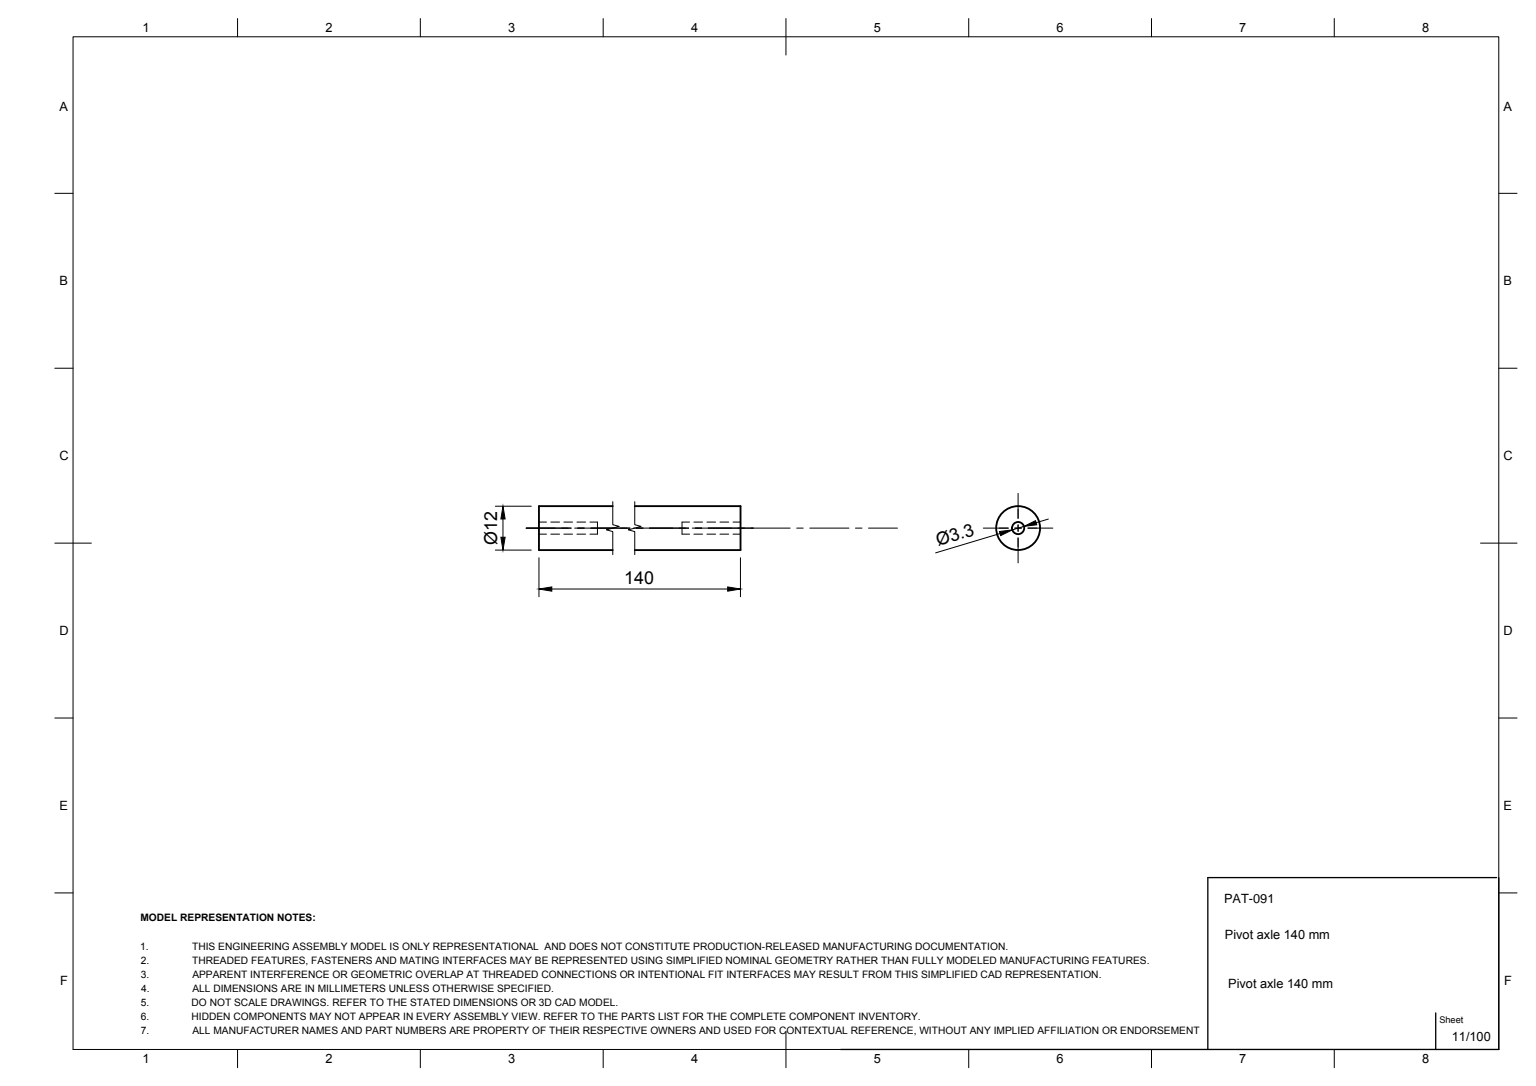
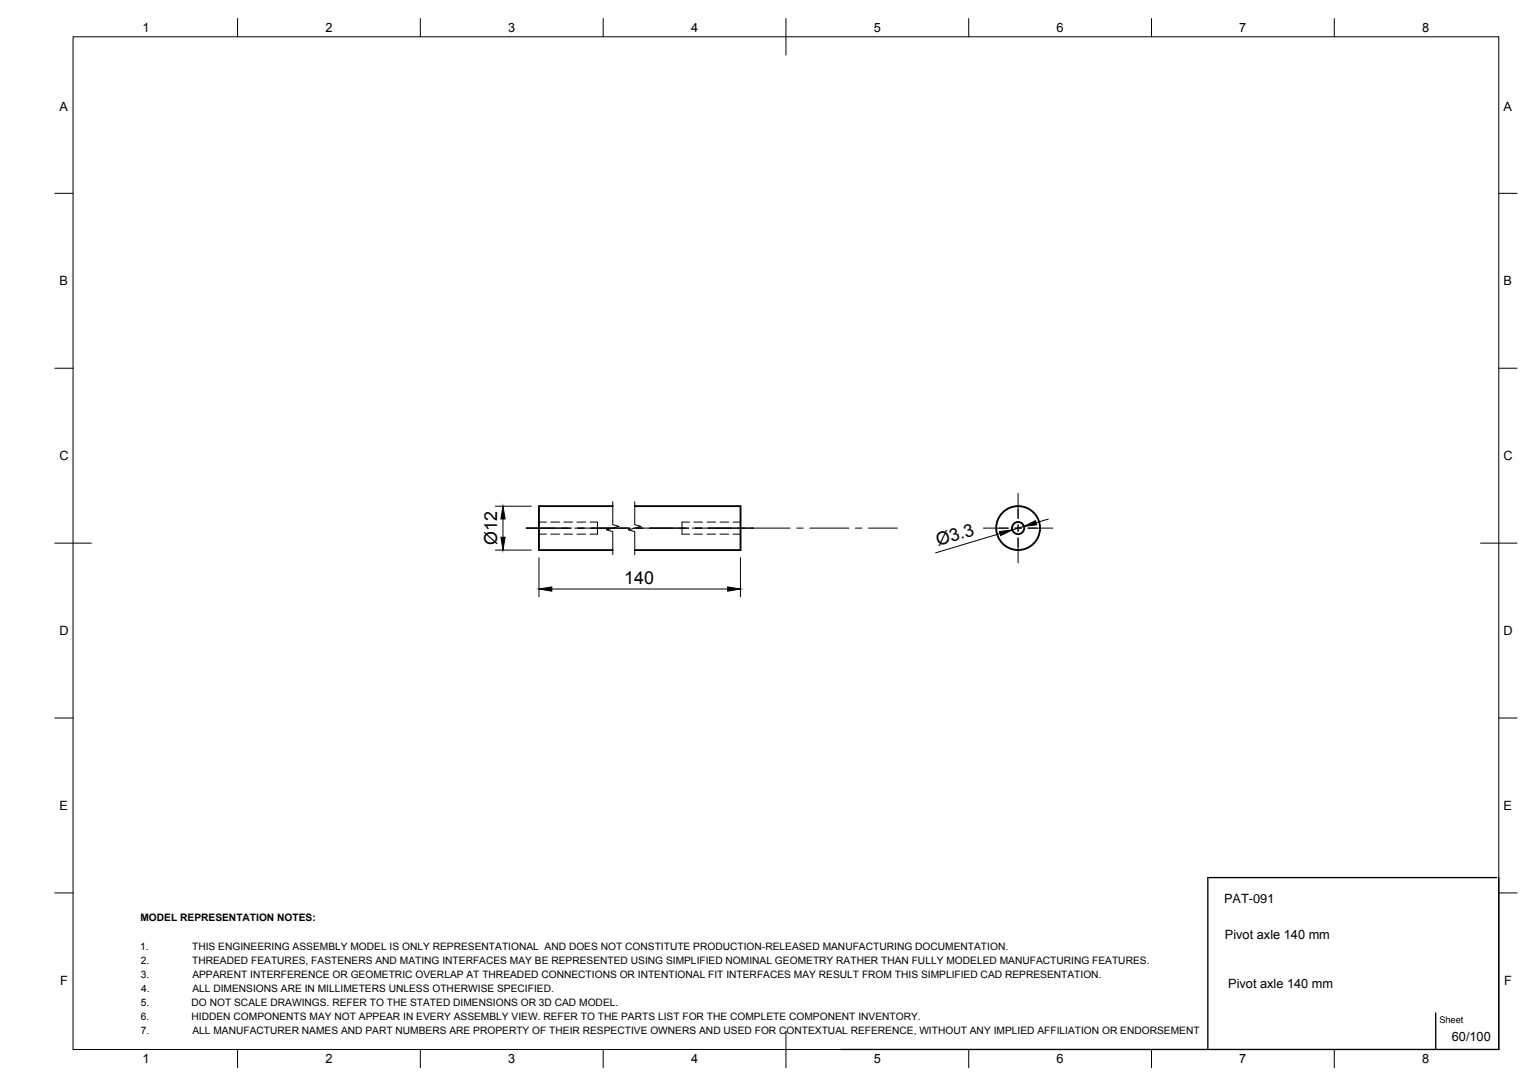
ISO-10303-21;
HEADER;
/* Generated by software containing ST-Developer
 * from STEP Tools, Inc. (www.steptools.com) 
 */

FILE_DESCRIPTION(
/* description */ ('PAT-091'),
/* implementation_level */ '2;1');

FILE_NAME(
/* name */ 'Pivot axle 140 mm.step',
/* time_stamp */ '2026-10-27T15:34:44-07:00',
/* author */ (''),
/* organization */ (''),
/* preprocessor_version */ 'ST-DEVELOPER v20.2',
/* originating_system */ 'Autodesk Translation Framework v15.17.0.0',
/* authorisation */ '');

FILE_SCHEMA (('AUTOMOTIVE_DESIGN { 1 0 10303 214 3 1 1 }'));
ENDSEC;

DATA;
#10=MECHANICAL_DESIGN_GEOMETRIC_PRESENTATION_REPRESENTATION('',(#982),#25100);
#762=SHAPE_REPRESENTATION_RELATIONSHIP('SRR','None',#25523,#872);
#872=ADVANCED_BREP_SHAPE_REPRESENTATION('',(#1106),#24993);
#982=STYLED_ITEM('',(#26191),#1106);
#1106=MANIFOLD_SOLID_BREP('Body1',#13259);
#1321=FACE_BOUND('',#3108,.T.);
#1322=FACE_BOUND('',#3110,.T.);
#1694=PLANE('',#14839);
#1695=PLANE('',#14843);
#1696=PLANE('',#14847);
#1697=PLANE('',#14848);
#2178=FACE_OUTER_BOUND('',#3102,.T.);
#2179=FACE_OUTER_BOUND('',#3103,.T.);
#2180=FACE_OUTER_BOUND('',#3104,.T.);
#2181=FACE_OUTER_BOUND('',#3105,.T.);
#2182=FACE_OUTER_BOUND('',#3106,.T.);
#2183=FACE_OUTER_BOUND('',#3107,.T.);
#2184=FACE_OUTER_BOUND('',#3109,.T.);
#3102=EDGE_LOOP('',(#9506,#9507,#9508,#9509));
#3103=EDGE_LOOP('',(#9510));
#3104=EDGE_LOOP('',(#9511,#9512,#9513,#9514));
#3105=EDGE_LOOP('',(#9515));
#3106=EDGE_LOOP('',(#9516,#9517,#9518,#9519));
#3107=EDGE_LOOP('',(#9520));
#3108=EDGE_LOOP('',(#9521));
#3109=EDGE_LOOP('',(#9522));
#3110=EDGE_LOOP('',(#9523));
#4269=LINE('',#21552,#5009);
#4270=LINE('',#21559,#5010);
#4271=LINE('',#21566,#5011);
#5009=VECTOR('',#17119,0.165);
#5010=VECTOR('',#17128,0.165);
#5011=VECTOR('',#17137,0.6);
#5726=CIRCLE('',#14837,0.165);
#5727=CIRCLE('',#14838,0.165);
#5728=CIRCLE('',#14841,0.165);
#5729=CIRCLE('',#14842,0.165);
#5730=CIRCLE('',#14845,0.6);
#5731=CIRCLE('',#14846,0.6);
#6561=VERTEX_POINT('',#21549);
#6562=VERTEX_POINT('',#21551);
#6563=VERTEX_POINT('',#21556);
#6564=VERTEX_POINT('',#21558);
#6565=VERTEX_POINT('',#21563);
#6566=VERTEX_POINT('',#21565);
#7688=EDGE_CURVE('',#6561,#6561,#5726,.T.);
#7689=EDGE_CURVE('',#6561,#6562,#4269,.T.);
#7690=EDGE_CURVE('',#6562,#6562,#5727,.T.);
#7691=EDGE_CURVE('',#6563,#6563,#5728,.T.);
#7692=EDGE_CURVE('',#6563,#6564,#4270,.T.);
#7693=EDGE_CURVE('',#6564,#6564,#5729,.T.);
#7694=EDGE_CURVE('',#6565,#6565,#5730,.T.);
#7695=EDGE_CURVE('',#6565,#6566,#4271,.T.);
#7696=EDGE_CURVE('',#6566,#6566,#5731,.T.);
#9506=ORIENTED_EDGE('',*,*,#7688,.F.);
#9507=ORIENTED_EDGE('',*,*,#7689,.T.);
#9508=ORIENTED_EDGE('',*,*,#7690,.F.);
#9509=ORIENTED_EDGE('',*,*,#7689,.F.);
#9510=ORIENTED_EDGE('',*,*,#7688,.T.);
#9511=ORIENTED_EDGE('',*,*,#7691,.F.);
#9512=ORIENTED_EDGE('',*,*,#7692,.T.);
#9513=ORIENTED_EDGE('',*,*,#7693,.T.);
#9514=ORIENTED_EDGE('',*,*,#7692,.F.);
#9515=ORIENTED_EDGE('',*,*,#7693,.F.);
#9516=ORIENTED_EDGE('',*,*,#7694,.F.);
#9517=ORIENTED_EDGE('',*,*,#7695,.T.);
#9518=ORIENTED_EDGE('',*,*,#7696,.T.);
#9519=ORIENTED_EDGE('',*,*,#7695,.F.);
#9520=ORIENTED_EDGE('',*,*,#7694,.T.);
#9521=ORIENTED_EDGE('',*,*,#7690,.T.);
#9522=ORIENTED_EDGE('',*,*,#7696,.F.);
#9523=ORIENTED_EDGE('',*,*,#7691,.T.);
#12135=CYLINDRICAL_SURFACE('',#14836,0.165);
#12136=CYLINDRICAL_SURFACE('',#14840,0.165);
#12137=CYLINDRICAL_SURFACE('',#14844,0.6);
#12545=ADVANCED_FACE('',(#2178),#12135,.F.);
#12546=ADVANCED_FACE('',(#2179),#1694,.T.);
#12547=ADVANCED_FACE('',(#2180),#12136,.F.);
#12548=ADVANCED_FACE('',(#2181),#1695,.F.);
#12549=ADVANCED_FACE('',(#2182),#12137,.T.);
#12550=ADVANCED_FACE('',(#2183,#1321),#1696,.T.);
#12551=ADVANCED_FACE('',(#2184,#1322),#1697,.F.);
#13259=CLOSED_SHELL('',(#12545,#12546,#12547,#12548,#12549,#12550,#12551));
#14835=AXIS2_PLACEMENT_3D('',#21547,#17113,#17114);
#14836=AXIS2_PLACEMENT_3D('',#21548,#17115,#17116);
#14837=AXIS2_PLACEMENT_3D('',#21550,#17117,#17118);
#14838=AXIS2_PLACEMENT_3D('',#21553,#17120,#17121);
#14839=AXIS2_PLACEMENT_3D('',#21554,#17122,#17123);
#14840=AXIS2_PLACEMENT_3D('',#21555,#17124,#17125);
#14841=AXIS2_PLACEMENT_3D('',#21557,#17126,#17127);
#14842=AXIS2_PLACEMENT_3D('',#21560,#17129,#17130);
#14843=AXIS2_PLACEMENT_3D('',#21561,#17131,#17132);
#14844=AXIS2_PLACEMENT_3D('',#21562,#17133,#17134);
#14845=AXIS2_PLACEMENT_3D('',#21564,#17135,#17136);
#14846=AXIS2_PLACEMENT_3D('',#21567,#17138,#17139);
#14847=AXIS2_PLACEMENT_3D('',#21568,#17140,#17141);
#14848=AXIS2_PLACEMENT_3D('',#21569,#17142,#17143);
#17113=DIRECTION('axis',(0.,0.,1.));
#17114=DIRECTION('refdir',(1.,0.,0.));
#17115=DIRECTION('center_axis',(0.,1.,0.));
#17116=DIRECTION('ref_axis',(1.,0.,0.));
#17117=DIRECTION('center_axis',(0.,1.,0.));
#17118=DIRECTION('ref_axis',(1.,0.,0.));
#17119=DIRECTION('',(0.,1.,0.));
#17120=DIRECTION('center_axis',(0.,-1.,0.));
#17121=DIRECTION('ref_axis',(1.,0.,0.));
#17122=DIRECTION('center_axis',(0.,1.,0.));
#17123=DIRECTION('ref_axis',(1.,0.,0.));
#17124=DIRECTION('center_axis',(0.,1.,0.));
#17125=DIRECTION('ref_axis',(1.,0.,0.));
#17126=DIRECTION('center_axis',(0.,1.,0.));
#17127=DIRECTION('ref_axis',(1.,0.,0.));
#17128=DIRECTION('',(0.,1.,0.));
#17129=DIRECTION('center_axis',(0.,1.,0.));
#17130=DIRECTION('ref_axis',(1.,0.,0.));
#17131=DIRECTION('center_axis',(0.,1.,0.));
#17132=DIRECTION('ref_axis',(1.,0.,0.));
#17133=DIRECTION('center_axis',(0.,1.,0.));
#17134=DIRECTION('ref_axis',(1.,0.,0.));
#17135=DIRECTION('center_axis',(0.,1.,0.));
#17136=DIRECTION('ref_axis',(1.,0.,0.));
#17137=DIRECTION('',(0.,-1.,0.));
#17138=DIRECTION('center_axis',(0.,1.,0.));
#17139=DIRECTION('ref_axis',(1.,0.,0.));
#17140=DIRECTION('center_axis',(0.,1.,0.));
#17141=DIRECTION('ref_axis',(1.,0.,0.));
#17142=DIRECTION('center_axis',(0.,1.,0.));
#17143=DIRECTION('ref_axis',(1.,0.,0.));
#21547=CARTESIAN_POINT('',(0.,0.,0.));
#21548=CARTESIAN_POINT('Origin',(0.,4.9,3.));
#21549=CARTESIAN_POINT('',(-0.165,4.9,3.));
#21550=CARTESIAN_POINT('Origin',(0.,4.9,3.));
#21551=CARTESIAN_POINT('',(-0.165,6.5,3.));
#21552=CARTESIAN_POINT('',(-0.165,4.9,3.));
#21553=CARTESIAN_POINT('Origin',(0.,6.5,3.));
#21554=CARTESIAN_POINT('Origin',(0.,4.9,3.));
#21555=CARTESIAN_POINT('Origin',(0.,-7.6,3.));
#21556=CARTESIAN_POINT('',(-0.165,-7.5,3.));
#21557=CARTESIAN_POINT('Origin',(0.,-7.5,3.));
#21558=CARTESIAN_POINT('',(-0.165,-5.9,3.));
#21559=CARTESIAN_POINT('',(-0.165,-7.6,3.));
#21560=CARTESIAN_POINT('Origin',(0.,-5.9,3.));
#21561=CARTESIAN_POINT('Origin',(0.,-5.9,3.));
#21562=CARTESIAN_POINT('Origin',(0.,-7.5,3.));
#21563=CARTESIAN_POINT('',(-0.6,6.5,3.));
#21564=CARTESIAN_POINT('Origin',(0.,6.5,3.));
#21565=CARTESIAN_POINT('',(-0.6,-7.5,3.));
#21566=CARTESIAN_POINT('',(-0.6,-7.5,3.));
#21567=CARTESIAN_POINT('Origin',(0.,-7.5,3.));
#21568=CARTESIAN_POINT('Origin',(0.,6.5,3.));
#21569=CARTESIAN_POINT('Origin',(0.,-7.5,3.));
#24872=UNCERTAINTY_MEASURE_WITH_UNIT(LENGTH_MEASURE(0.001),#25101,
'DISTANCE_ACCURACY_VALUE',
'Maximum model space distance between geometric entities at asserted c
onnectivities');
#24979=UNCERTAINTY_MEASURE_WITH_UNIT(LENGTH_MEASURE(0.001),#25101,
'DISTANCE_ACCURACY_VALUE',
'Maximum model space distance between geometric entities at asserted c
onnectivities');
#24993=(
GEOMETRIC_REPRESENTATION_CONTEXT(3)
GLOBAL_UNCERTAINTY_ASSIGNED_CONTEXT((#24872))
GLOBAL_UNIT_ASSIGNED_CONTEXT((#25101,#25103,#25104))
REPRESENTATION_CONTEXT('','3D')
);
#25100=(
GEOMETRIC_REPRESENTATION_CONTEXT(3)
GLOBAL_UNCERTAINTY_ASSIGNED_CONTEXT((#24979))
GLOBAL_UNIT_ASSIGNED_CONTEXT((#25101,#25103,#25104))
REPRESENTATION_CONTEXT('','3D')
);
#25101=(
LENGTH_UNIT()
NAMED_UNIT(*)
SI_UNIT(.CENTI.,.METRE.)
);
#25103=(
NAMED_UNIT(*)
PLANE_ANGLE_UNIT()
SI_UNIT($,.RADIAN.)
);
#25104=(
NAMED_UNIT(*)
SI_UNIT($,.STERADIAN.)
SOLID_ANGLE_UNIT()
);
#25118=SHAPE_DEFINITION_REPRESENTATION(#25238,#25523);
#25238=PRODUCT_DEFINITION_SHAPE('',$,#25644);
#25523=SHAPE_REPRESENTATION('',(#14835),#24993);
#25630=PRODUCT_DEFINITION_CONTEXT('part definition',#25992,'design');
#25644=PRODUCT_DEFINITION('Pivot axle 140 mm','Pivot axle 140 mm',#25764,
#25630);
#25764=PRODUCT_DEFINITION_FORMATION('',$,#26007);
#25992=APPLICATION_CONTEXT(
'Core Data for Automotive Mechanical Design Process');
#25993=PRODUCT_CONTEXT('part definition',#25992,'mechanical');
#26007=PRODUCT('Pivot axle 140 mm','Pivot axle 140 mm',
'Pivot axle 140 mm',(#25993));
#26185=COLOUR_RGB('Grey',0.48,0.52,0.57);
#26186=FILL_AREA_STYLE_COLOUR('',#26185);
#26187=FILL_AREA_STYLE('',(#26186));
#26188=SURFACE_STYLE_FILL_AREA(#26187);
#26189=SURFACE_SIDE_STYLE('',(#26188));
#26190=SURFACE_STYLE_USAGE(.BOTH.,#26189);
#26191=PRESENTATION_STYLE_ASSIGNMENT((#26190));
ENDSEC;
END-ISO-10303-21;
